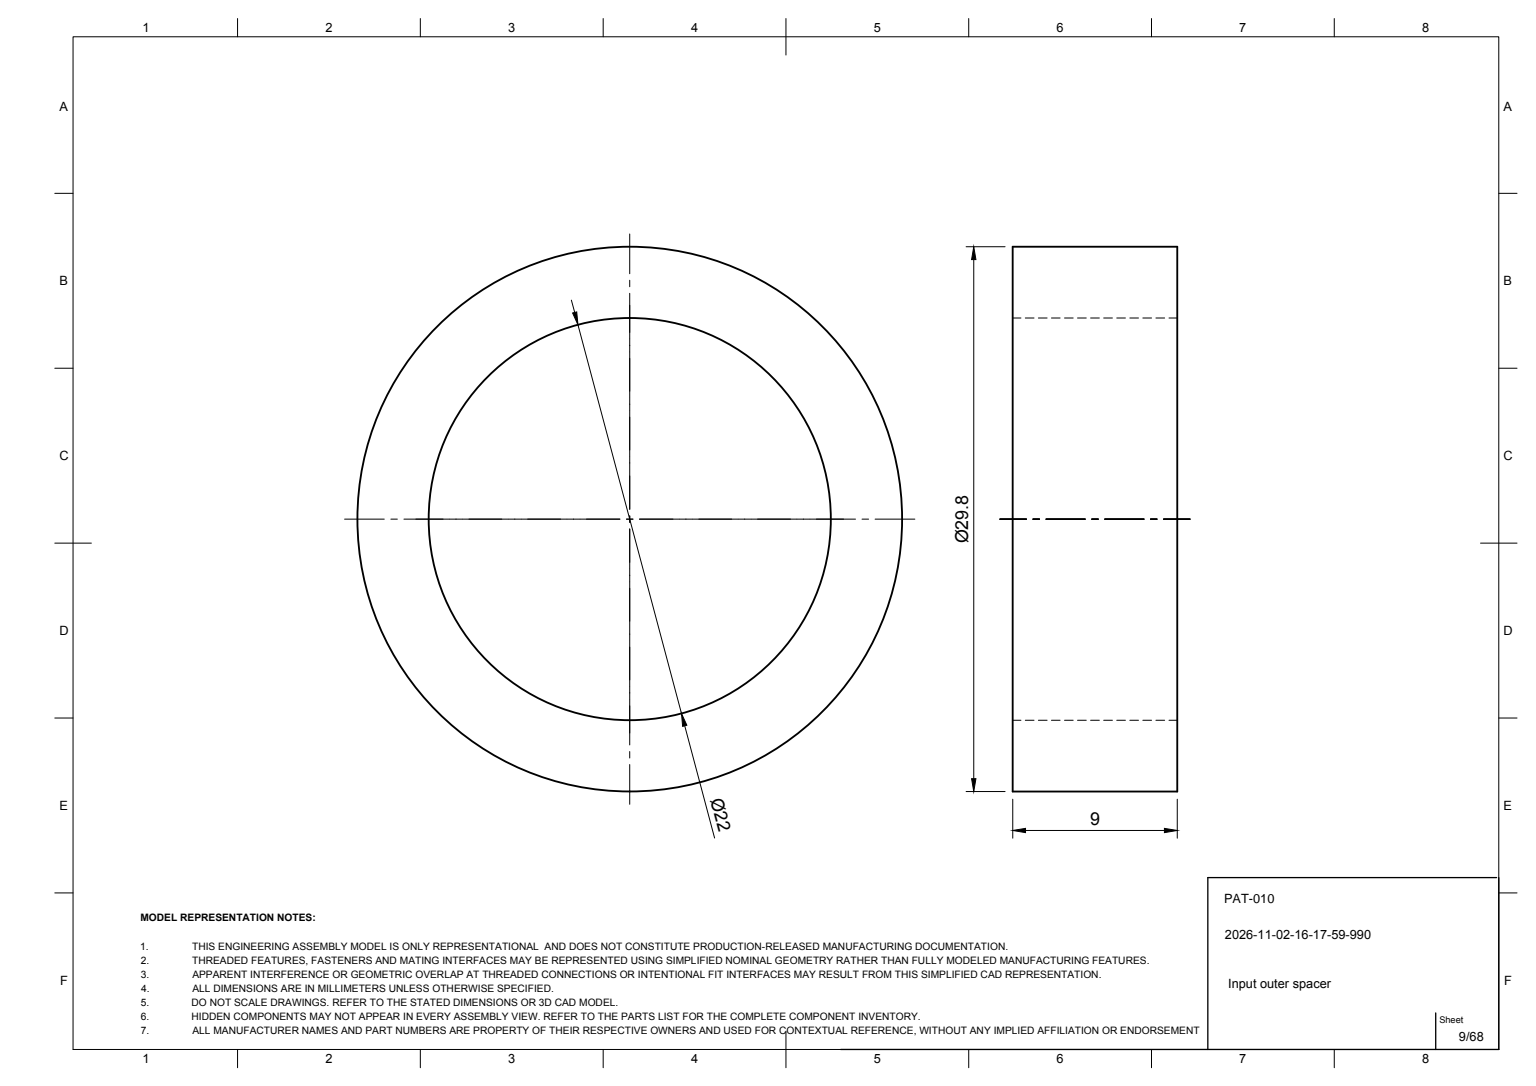
ISO-10303-21;
HEADER;
/* Generated by software containing ST-Developer
 * from STEP Tools, Inc. (www.steptools.com) 
 */

FILE_DESCRIPTION(
/* description */ ('Belt conveyor head drive unit'),
/* implementation_level */ '2;1');

FILE_NAME(
/* name */ 'Input outer spacer.step',
/* time_stamp */ '2026-10-28T03:26:19-07:00',
/* author */ (''),
/* organization */ (''),
/* preprocessor_version */ 'ST-DEVELOPER v20.2',
/* originating_system */ 'Autodesk Translation Framework v15.17.0.0',
/* authorisation */ '');

FILE_SCHEMA (('AUTOMOTIVE_DESIGN { 1 0 10303 214 3 1 1 }'));
ENDSEC;

DATA;
#10=MECHANICAL_DESIGN_GEOMETRIC_PRESENTATION_REPRESENTATION('',(#851),#27069);
#713=SHAPE_REPRESENTATION_RELATIONSHIP('SRR','None',#27357,#782);
#782=ADVANCED_BREP_SHAPE_REPRESENTATION('',(#936),#26999);
#851=STYLED_ITEM('',(#27790),#936);
#936=MANIFOLD_SOLID_BREP('Body1',#13716);
#1050=FACE_BOUND('',#2555,.T.);
#1051=FACE_BOUND('',#2557,.T.);
#1327=PLANE('',#14722);
#1328=PLANE('',#14723);
#1714=FACE_OUTER_BOUND('',#2552,.T.);
#1715=FACE_OUTER_BOUND('',#2553,.T.);
#1716=FACE_OUTER_BOUND('',#2554,.T.);
#1717=FACE_OUTER_BOUND('',#2556,.T.);
#2552=EDGE_LOOP('',(#9324,#9325,#9326,#9327));
#2553=EDGE_LOOP('',(#9328,#9329,#9330,#9331));
#2554=EDGE_LOOP('',(#9332));
#2555=EDGE_LOOP('',(#9333));
#2556=EDGE_LOOP('',(#9334));
#2557=EDGE_LOOP('',(#9335));
#3615=LINE('',#21367,#4407);
#3616=LINE('',#21373,#4408);
#4407=VECTOR('',#16863,1.1);
#4408=VECTOR('',#16870,1.49);
#5148=CIRCLE('',#14717,1.1);
#5149=CIRCLE('',#14718,1.1);
#5150=CIRCLE('',#14720,1.49);
#5151=CIRCLE('',#14721,1.49);
#6075=VERTEX_POINT('',#21364);
#6076=VERTEX_POINT('',#21366);
#6077=VERTEX_POINT('',#21370);
#6078=VERTEX_POINT('',#21372);
#7354=EDGE_CURVE('',#6075,#6075,#5148,.T.);
#7355=EDGE_CURVE('',#6075,#6076,#3615,.T.);
#7356=EDGE_CURVE('',#6076,#6076,#5149,.T.);
#7357=EDGE_CURVE('',#6077,#6077,#5150,.T.);
#7358=EDGE_CURVE('',#6077,#6078,#3616,.T.);
#7359=EDGE_CURVE('',#6078,#6078,#5151,.T.);
#9324=ORIENTED_EDGE('',*,*,#7354,.F.);
#9325=ORIENTED_EDGE('',*,*,#7355,.T.);
#9326=ORIENTED_EDGE('',*,*,#7356,.T.);
#9327=ORIENTED_EDGE('',*,*,#7355,.F.);
#9328=ORIENTED_EDGE('',*,*,#7357,.F.);
#9329=ORIENTED_EDGE('',*,*,#7358,.T.);
#9330=ORIENTED_EDGE('',*,*,#7359,.T.);
#9331=ORIENTED_EDGE('',*,*,#7358,.F.);
#9332=ORIENTED_EDGE('',*,*,#7357,.T.);
#9333=ORIENTED_EDGE('',*,*,#7354,.T.);
#9334=ORIENTED_EDGE('',*,*,#7359,.F.);
#9335=ORIENTED_EDGE('',*,*,#7356,.F.);
#12563=CYLINDRICAL_SURFACE('',#14716,1.1);
#12564=CYLINDRICAL_SURFACE('',#14719,1.49);
#12993=ADVANCED_FACE('',(#1714),#12563,.F.);
#12994=ADVANCED_FACE('',(#1715),#12564,.T.);
#12995=ADVANCED_FACE('',(#1716,#1050),#1327,.T.);
#12996=ADVANCED_FACE('',(#1717,#1051),#1328,.F.);
#13716=CLOSED_SHELL('',(#12993,#12994,#12995,#12996));
#14715=AXIS2_PLACEMENT_3D('',#21362,#16857,#16858);
#14716=AXIS2_PLACEMENT_3D('',#21363,#16859,#16860);
#14717=AXIS2_PLACEMENT_3D('',#21365,#16861,#16862);
#14718=AXIS2_PLACEMENT_3D('',#21368,#16864,#16865);
#14719=AXIS2_PLACEMENT_3D('',#21369,#16866,#16867);
#14720=AXIS2_PLACEMENT_3D('',#21371,#16868,#16869);
#14721=AXIS2_PLACEMENT_3D('',#21374,#16871,#16872);
#14722=AXIS2_PLACEMENT_3D('',#21375,#16873,#16874);
#14723=AXIS2_PLACEMENT_3D('',#21376,#16875,#16876);
#16857=DIRECTION('axis',(0.,0.,1.));
#16858=DIRECTION('refdir',(1.,0.,0.));
#16859=DIRECTION('center_axis',(0.,1.,0.));
#16860=DIRECTION('ref_axis',(1.,0.,0.));
#16861=DIRECTION('center_axis',(0.,-1.,0.));
#16862=DIRECTION('ref_axis',(1.,0.,0.));
#16863=DIRECTION('',(0.,-1.,0.));
#16864=DIRECTION('center_axis',(0.,-1.,0.));
#16865=DIRECTION('ref_axis',(1.,0.,0.));
#16866=DIRECTION('center_axis',(0.,1.,0.));
#16867=DIRECTION('ref_axis',(1.,0.,0.));
#16868=DIRECTION('center_axis',(0.,1.,0.));
#16869=DIRECTION('ref_axis',(1.,0.,0.));
#16870=DIRECTION('',(0.,-1.,0.));
#16871=DIRECTION('center_axis',(0.,1.,0.));
#16872=DIRECTION('ref_axis',(1.,0.,0.));
#16873=DIRECTION('center_axis',(0.,1.,0.));
#16874=DIRECTION('ref_axis',(1.,0.,0.));
#16875=DIRECTION('center_axis',(0.,1.,0.));
#16876=DIRECTION('ref_axis',(1.,0.,0.));
#21362=CARTESIAN_POINT('',(0.,0.,0.));
#21363=CARTESIAN_POINT('Origin',(0.,-0.45,7.));
#21364=CARTESIAN_POINT('',(-1.1,0.45,7.));
#21365=CARTESIAN_POINT('Origin',(0.,0.45,7.));
#21366=CARTESIAN_POINT('',(-1.1,-0.45,7.));
#21367=CARTESIAN_POINT('',(-1.1,-0.45,7.));
#21368=CARTESIAN_POINT('Origin',(0.,-0.45,7.));
#21369=CARTESIAN_POINT('Origin',(0.,-0.45,7.));
#21370=CARTESIAN_POINT('',(-1.49,0.45,7.));
#21371=CARTESIAN_POINT('Origin',(0.,0.45,7.));
#21372=CARTESIAN_POINT('',(-1.49,-0.45,7.));
#21373=CARTESIAN_POINT('',(-1.49,-0.45,7.));
#21374=CARTESIAN_POINT('Origin',(0.,-0.45,7.));
#21375=CARTESIAN_POINT('Origin',(0.,0.45,7.));
#21376=CARTESIAN_POINT('Origin',(0.,-0.45,7.));
#26922=UNCERTAINTY_MEASURE_WITH_UNIT(LENGTH_MEASURE(0.001),#27070,
'DISTANCE_ACCURACY_VALUE',
'Maximum model space distance between geometric entities at asserted c
onnectivities');
#26992=UNCERTAINTY_MEASURE_WITH_UNIT(LENGTH_MEASURE(0.001),#27070,
'DISTANCE_ACCURACY_VALUE',
'Maximum model space distance between geometric entities at asserted c
onnectivities');
#26999=(
GEOMETRIC_REPRESENTATION_CONTEXT(3)
GLOBAL_UNCERTAINTY_ASSIGNED_CONTEXT((#26922))
GLOBAL_UNIT_ASSIGNED_CONTEXT((#27070,#27072,#27073))
REPRESENTATION_CONTEXT('','3D')
);
#27069=(
GEOMETRIC_REPRESENTATION_CONTEXT(3)
GLOBAL_UNCERTAINTY_ASSIGNED_CONTEXT((#26992))
GLOBAL_UNIT_ASSIGNED_CONTEXT((#27070,#27072,#27073))
REPRESENTATION_CONTEXT('','3D')
);
#27070=(
LENGTH_UNIT()
NAMED_UNIT(*)
SI_UNIT(.CENTI.,.METRE.)
);
#27072=(
NAMED_UNIT(*)
PLANE_ANGLE_UNIT()
SI_UNIT($,.RADIAN.)
);
#27073=(
NAMED_UNIT(*)
SI_UNIT($,.STERADIAN.)
SOLID_ANGLE_UNIT()
);
#27080=SHAPE_DEFINITION_REPRESENTATION(#27156,#27357);
#27156=PRODUCT_DEFINITION_SHAPE('',$,#27434);
#27357=SHAPE_REPRESENTATION('',(#14715),#26999);
#27427=PRODUCT_DEFINITION_CONTEXT('part definition',#27657,'design');
#27434=PRODUCT_DEFINITION('Input outer spacer','Input outer spacer',#27510,
#27427);
#27510=PRODUCT_DEFINITION_FORMATION('',$,#27665);
#27657=APPLICATION_CONTEXT(
'Core Data for Automotive Mechanical Design Process');
#27658=PRODUCT_CONTEXT('part definition',#27657,'mechanical');
#27665=PRODUCT('Input outer spacer','Input outer spacer',
'Input outer spacer',(#27658));
#27784=COLOUR_RGB('Sky Blue',0.24,0.69,0.87);
#27785=FILL_AREA_STYLE_COLOUR('',#27784);
#27786=FILL_AREA_STYLE('',(#27785));
#27787=SURFACE_STYLE_FILL_AREA(#27786);
#27788=SURFACE_SIDE_STYLE('',(#27787));
#27789=SURFACE_STYLE_USAGE(.BOTH.,#27788);
#27790=PRESENTATION_STYLE_ASSIGNMENT((#27789));
ENDSEC;
END-ISO-10303-21;
